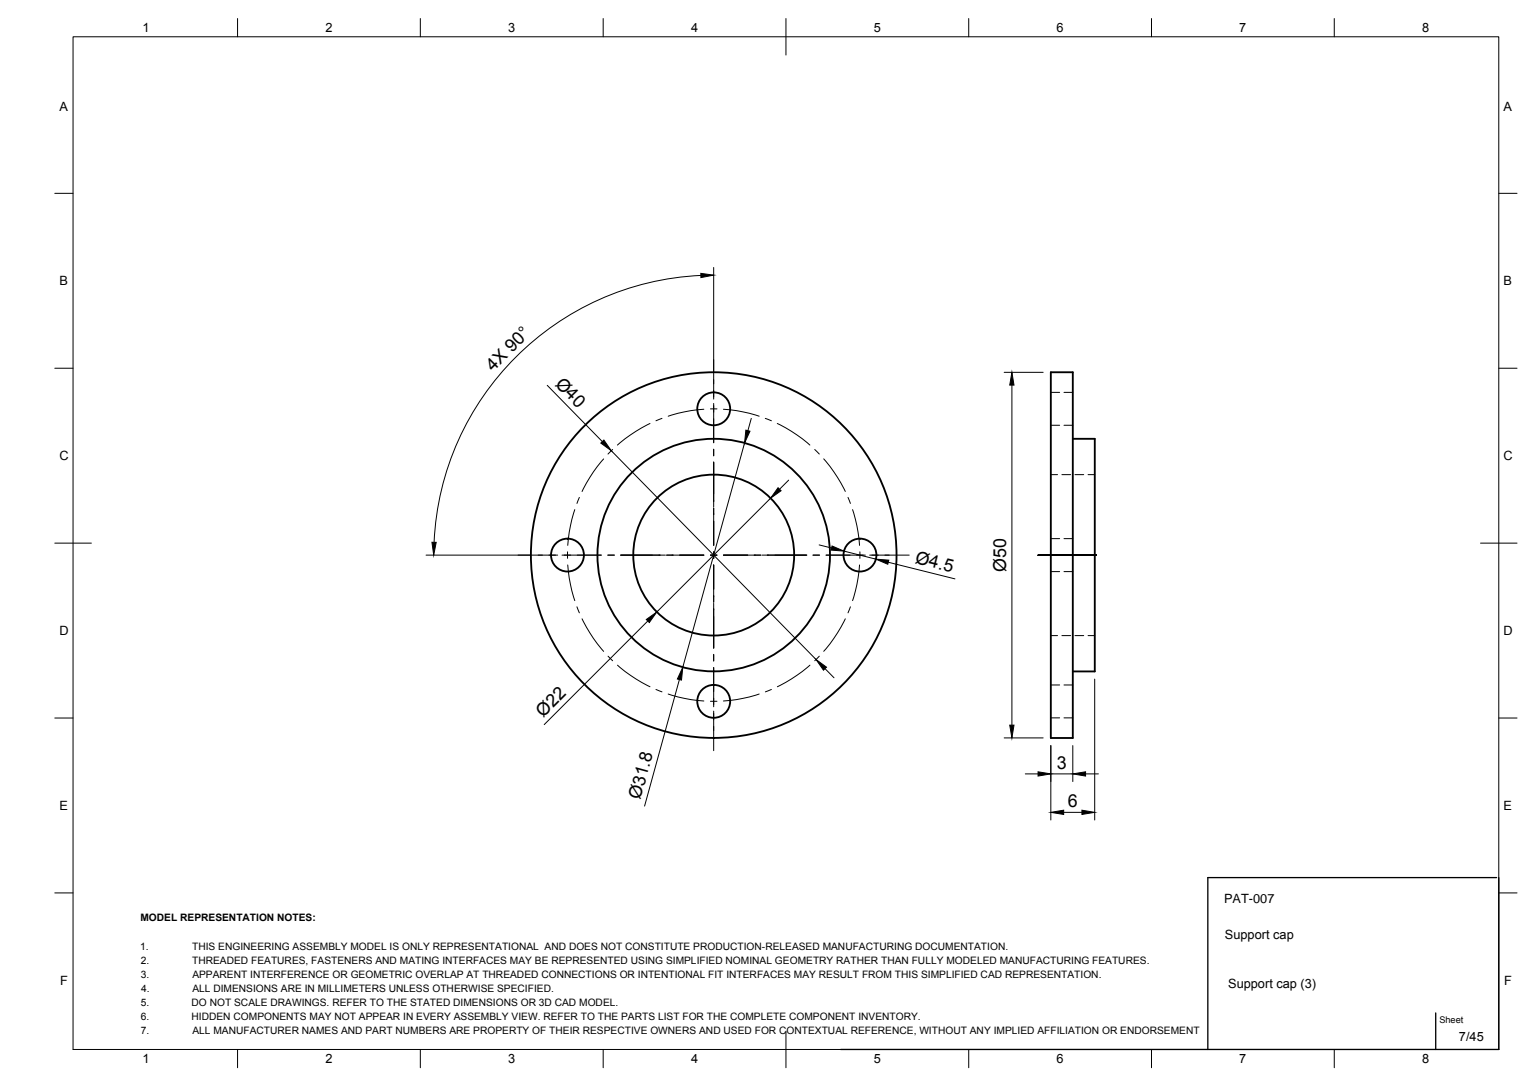
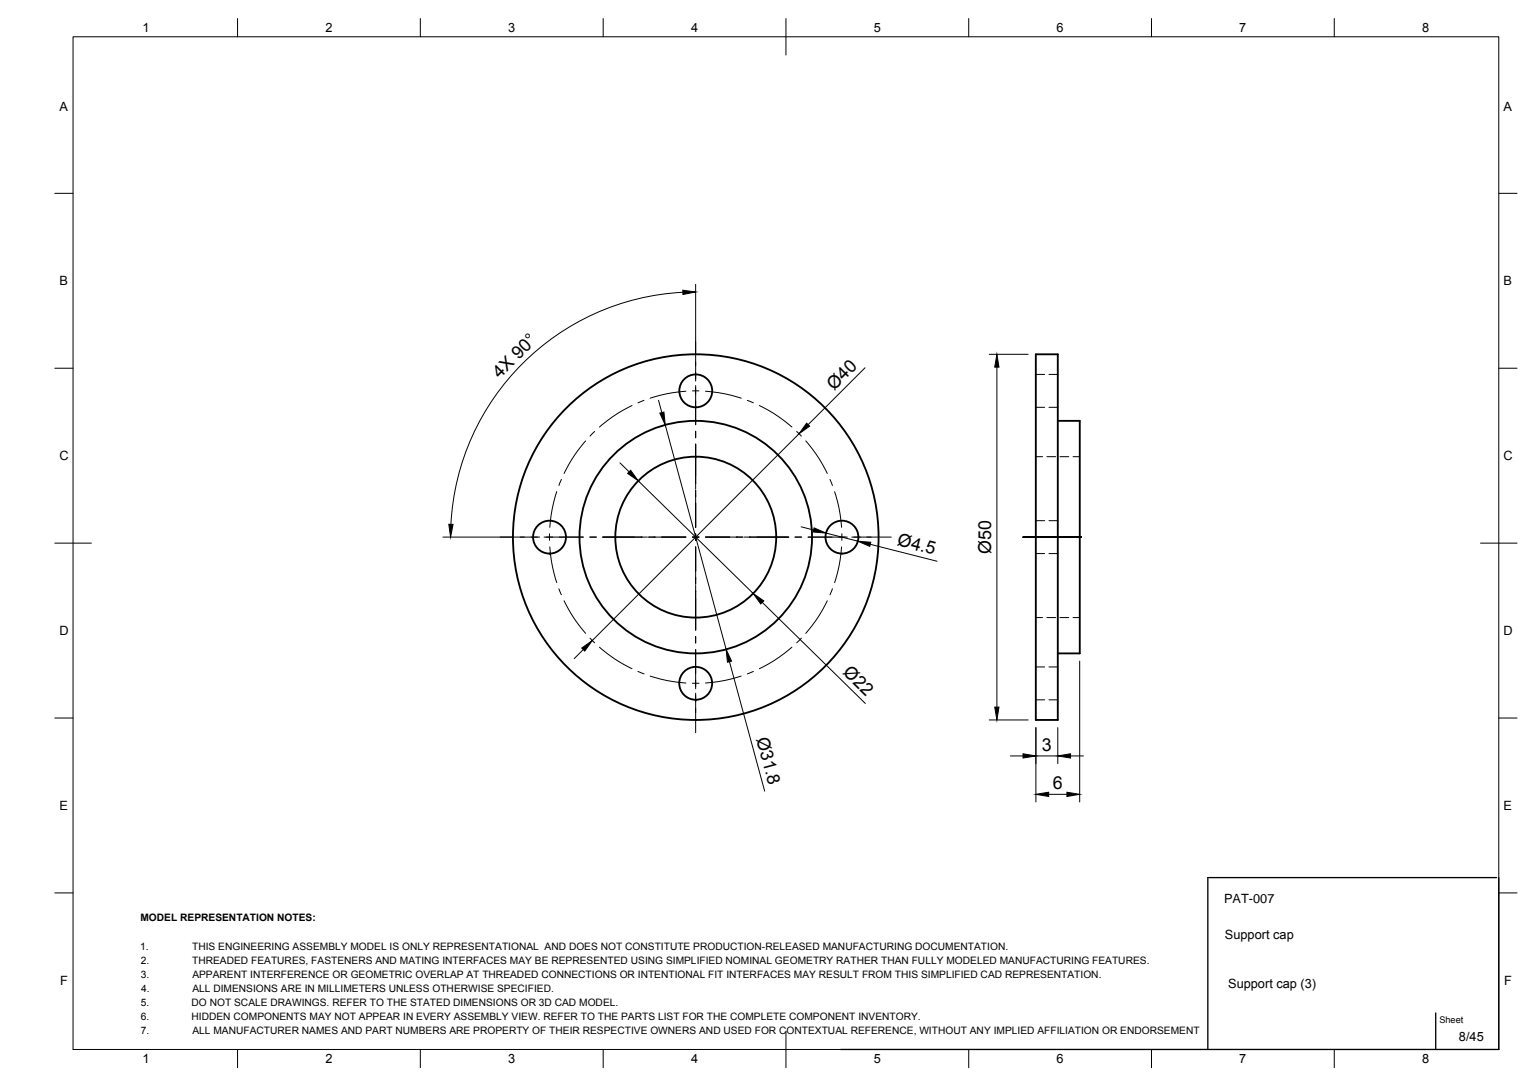
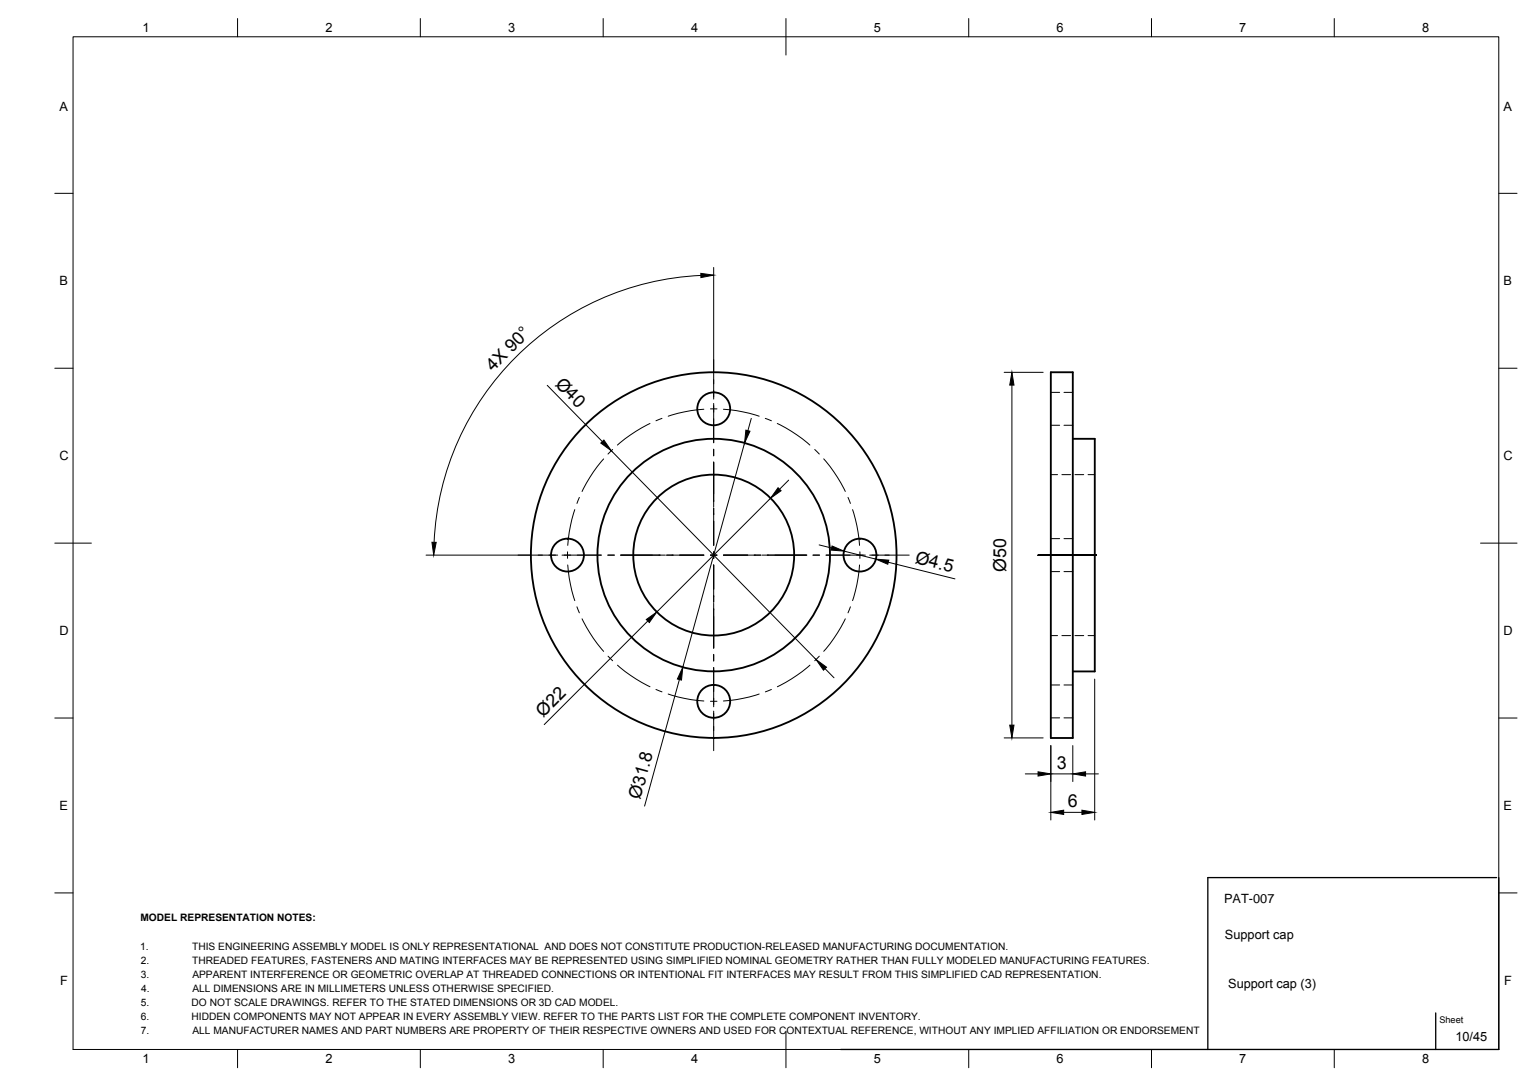
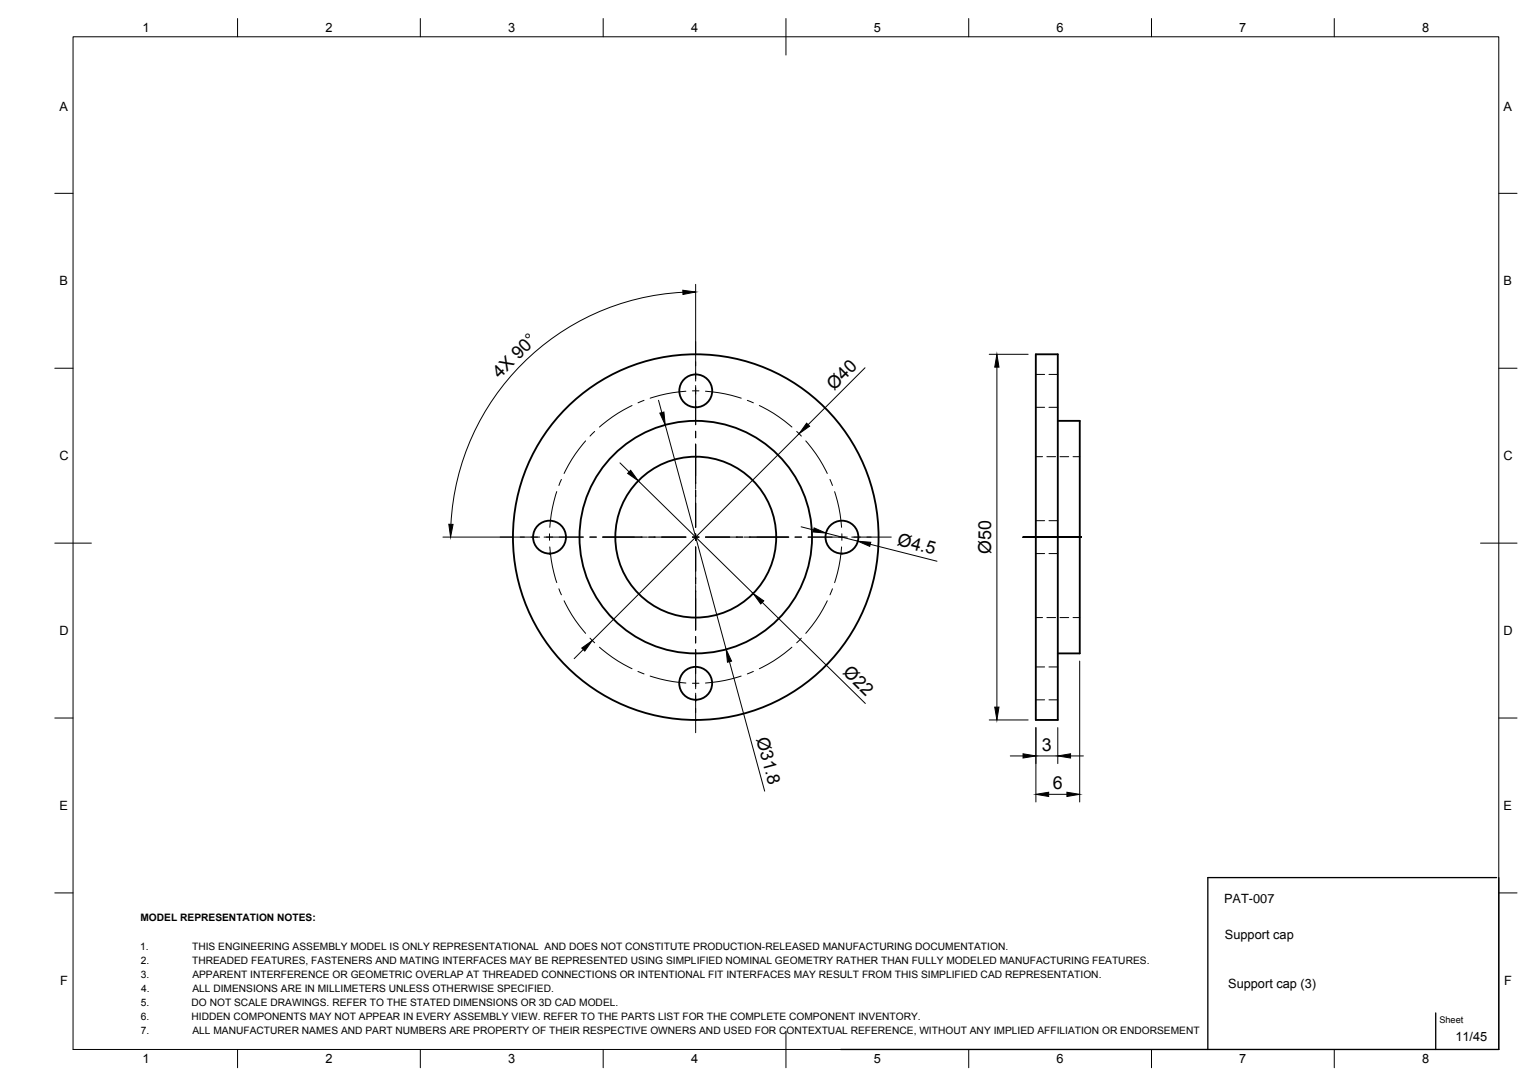
ISO-10303-21;
HEADER;
/* Generated by software containing ST-Developer
 * from STEP Tools, Inc. (www.steptools.com) 
 */

FILE_DESCRIPTION(
/* description */ ('Bearing friction torque test rig'),
/* implementation_level */ '2;1');

FILE_NAME(
/* name */ 'Support cap.step',
/* time_stamp */ '2026-10-28T03:24:04-07:00',
/* author */ (''),
/* organization */ (''),
/* preprocessor_version */ 'ST-DEVELOPER v20.2',
/* originating_system */ 'Autodesk Translation Framework v15.17.0.0',
/* authorisation */ '');

FILE_SCHEMA (('AUTOMOTIVE_DESIGN { 1 0 10303 214 3 1 1 }'));
ENDSEC;

DATA;
#10=MECHANICAL_DESIGN_GEOMETRIC_PRESENTATION_REPRESENTATION('',(#541),#14822);
#463=SHAPE_REPRESENTATION_RELATIONSHIP('SRR','None',#15002,#502);
#502=ADVANCED_BREP_SHAPE_REPRESENTATION('',(#595),#14782);
#541=STYLED_ITEM('',(#15277),#595);
#595=MANIFOLD_SOLID_BREP('Body1',#7657);
#684=FACE_BOUND('',#1629,.T.);
#685=FACE_BOUND('',#1633,.T.);
#686=FACE_BOUND('',#1634,.T.);
#687=FACE_BOUND('',#1635,.T.);
#688=FACE_BOUND('',#1636,.T.);
#689=FACE_BOUND('',#1637,.T.);
#690=FACE_BOUND('',#1639,.T.);
#691=FACE_BOUND('',#1640,.T.);
#692=FACE_BOUND('',#1641,.T.);
#693=FACE_BOUND('',#1642,.T.);
#694=FACE_BOUND('',#1643,.T.);
#891=PLANE('',#8249);
#892=PLANE('',#8256);
#893=PLANE('',#8257);
#1138=FACE_OUTER_BOUND('',#1623,.T.);
#1139=FACE_OUTER_BOUND('',#1624,.T.);
#1140=FACE_OUTER_BOUND('',#1625,.T.);
#1141=FACE_OUTER_BOUND('',#1626,.T.);
#1142=FACE_OUTER_BOUND('',#1627,.T.);
#1143=FACE_OUTER_BOUND('',#1628,.T.);
#1144=FACE_OUTER_BOUND('',#1630,.T.);
#1145=FACE_OUTER_BOUND('',#1631,.T.);
#1146=FACE_OUTER_BOUND('',#1632,.T.);
#1147=FACE_OUTER_BOUND('',#1638,.T.);
#1623=EDGE_LOOP('',(#5346,#5347,#5348,#5349));
#1624=EDGE_LOOP('',(#5350,#5351,#5352,#5353));
#1625=EDGE_LOOP('',(#5354,#5355,#5356,#5357));
#1626=EDGE_LOOP('',(#5358,#5359,#5360,#5361));
#1627=EDGE_LOOP('',(#5362,#5363,#5364,#5365));
#1628=EDGE_LOOP('',(#5366));
#1629=EDGE_LOOP('',(#5367));
#1630=EDGE_LOOP('',(#5368,#5369,#5370,#5371));
#1631=EDGE_LOOP('',(#5372,#5373,#5374,#5375));
#1632=EDGE_LOOP('',(#5376));
#1633=EDGE_LOOP('',(#5377));
#1634=EDGE_LOOP('',(#5378));
#1635=EDGE_LOOP('',(#5379));
#1636=EDGE_LOOP('',(#5380));
#1637=EDGE_LOOP('',(#5381));
#1638=EDGE_LOOP('',(#5382));
#1639=EDGE_LOOP('',(#5383));
#1640=EDGE_LOOP('',(#5384));
#1641=EDGE_LOOP('',(#5385));
#1642=EDGE_LOOP('',(#5386));
#1643=EDGE_LOOP('',(#5387));
#2270=LINE('',#11871,#2714);
#2271=LINE('',#11877,#2715);
#2272=LINE('',#11883,#2716);
#2273=LINE('',#11889,#2717);
#2274=LINE('',#11895,#2718);
#2275=LINE('',#11902,#2719);
#2276=LINE('',#11908,#2720);
#2714=VECTOR('',#9405,0.225);
#2715=VECTOR('',#9412,0.225);
#2716=VECTOR('',#9419,0.225);
#2717=VECTOR('',#9426,0.225);
#2718=VECTOR('',#9433,1.59);
#2719=VECTOR('',#9442,1.1);
#2720=VECTOR('',#9449,2.5);
#3152=CIRCLE('',#8235,0.225);
#3153=CIRCLE('',#8236,0.225);
#3154=CIRCLE('',#8238,0.225);
#3155=CIRCLE('',#8239,0.225);
#3156=CIRCLE('',#8241,0.225);
#3157=CIRCLE('',#8242,0.225);
#3158=CIRCLE('',#8244,0.225);
#3159=CIRCLE('',#8245,0.225);
#3160=CIRCLE('',#8247,1.59);
#3161=CIRCLE('',#8248,1.59);
#3162=CIRCLE('',#8250,1.1);
#3163=CIRCLE('',#8252,1.1);
#3164=CIRCLE('',#8254,2.5);
#3165=CIRCLE('',#8255,2.5);
#3619=VERTEX_POINT('',#11868);
#3620=VERTEX_POINT('',#11870);
#3621=VERTEX_POINT('',#11874);
#3622=VERTEX_POINT('',#11876);
#3623=VERTEX_POINT('',#11880);
#3624=VERTEX_POINT('',#11882);
#3625=VERTEX_POINT('',#11886);
#3626=VERTEX_POINT('',#11888);
#3627=VERTEX_POINT('',#11892);
#3628=VERTEX_POINT('',#11894);
#3629=VERTEX_POINT('',#11898);
#3630=VERTEX_POINT('',#11901);
#3631=VERTEX_POINT('',#11905);
#3632=VERTEX_POINT('',#11907);
#4299=EDGE_CURVE('',#3619,#3619,#3152,.T.);
#4300=EDGE_CURVE('',#3619,#3620,#2270,.T.);
#4301=EDGE_CURVE('',#3620,#3620,#3153,.T.);
#4302=EDGE_CURVE('',#3621,#3621,#3154,.T.);
#4303=EDGE_CURVE('',#3621,#3622,#2271,.T.);
#4304=EDGE_CURVE('',#3622,#3622,#3155,.T.);
#4305=EDGE_CURVE('',#3623,#3623,#3156,.T.);
#4306=EDGE_CURVE('',#3623,#3624,#2272,.T.);
#4307=EDGE_CURVE('',#3624,#3624,#3157,.T.);
#4308=EDGE_CURVE('',#3625,#3625,#3158,.T.);
#4309=EDGE_CURVE('',#3625,#3626,#2273,.T.);
#4310=EDGE_CURVE('',#3626,#3626,#3159,.T.);
#4311=EDGE_CURVE('',#3627,#3627,#3160,.T.);
#4312=EDGE_CURVE('',#3627,#3628,#2274,.T.);
#4313=EDGE_CURVE('',#3628,#3628,#3161,.T.);
#4314=EDGE_CURVE('',#3629,#3629,#3162,.T.);
#4315=EDGE_CURVE('',#3629,#3630,#2275,.T.);
#4316=EDGE_CURVE('',#3630,#3630,#3163,.T.);
#4317=EDGE_CURVE('',#3631,#3631,#3164,.T.);
#4318=EDGE_CURVE('',#3631,#3632,#2276,.T.);
#4319=EDGE_CURVE('',#3632,#3632,#3165,.T.);
#5346=ORIENTED_EDGE('',*,*,#4299,.F.);
#5347=ORIENTED_EDGE('',*,*,#4300,.T.);
#5348=ORIENTED_EDGE('',*,*,#4301,.F.);
#5349=ORIENTED_EDGE('',*,*,#4300,.F.);
#5350=ORIENTED_EDGE('',*,*,#4302,.F.);
#5351=ORIENTED_EDGE('',*,*,#4303,.T.);
#5352=ORIENTED_EDGE('',*,*,#4304,.F.);
#5353=ORIENTED_EDGE('',*,*,#4303,.F.);
#5354=ORIENTED_EDGE('',*,*,#4305,.F.);
#5355=ORIENTED_EDGE('',*,*,#4306,.T.);
#5356=ORIENTED_EDGE('',*,*,#4307,.F.);
#5357=ORIENTED_EDGE('',*,*,#4306,.F.);
#5358=ORIENTED_EDGE('',*,*,#4308,.F.);
#5359=ORIENTED_EDGE('',*,*,#4309,.T.);
#5360=ORIENTED_EDGE('',*,*,#4310,.F.);
#5361=ORIENTED_EDGE('',*,*,#4309,.F.);
#5362=ORIENTED_EDGE('',*,*,#4311,.F.);
#5363=ORIENTED_EDGE('',*,*,#4312,.T.);
#5364=ORIENTED_EDGE('',*,*,#4313,.F.);
#5365=ORIENTED_EDGE('',*,*,#4312,.F.);
#5366=ORIENTED_EDGE('',*,*,#4311,.T.);
#5367=ORIENTED_EDGE('',*,*,#4314,.T.);
#5368=ORIENTED_EDGE('',*,*,#4314,.F.);
#5369=ORIENTED_EDGE('',*,*,#4315,.T.);
#5370=ORIENTED_EDGE('',*,*,#4316,.T.);
#5371=ORIENTED_EDGE('',*,*,#4315,.F.);
#5372=ORIENTED_EDGE('',*,*,#4317,.F.);
#5373=ORIENTED_EDGE('',*,*,#4318,.T.);
#5374=ORIENTED_EDGE('',*,*,#4319,.T.);
#5375=ORIENTED_EDGE('',*,*,#4318,.F.);
#5376=ORIENTED_EDGE('',*,*,#4317,.T.);
#5377=ORIENTED_EDGE('',*,*,#4313,.T.);
#5378=ORIENTED_EDGE('',*,*,#4310,.T.);
#5379=ORIENTED_EDGE('',*,*,#4307,.T.);
#5380=ORIENTED_EDGE('',*,*,#4304,.T.);
#5381=ORIENTED_EDGE('',*,*,#4301,.T.);
#5382=ORIENTED_EDGE('',*,*,#4319,.F.);
#5383=ORIENTED_EDGE('',*,*,#4316,.F.);
#5384=ORIENTED_EDGE('',*,*,#4308,.T.);
#5385=ORIENTED_EDGE('',*,*,#4305,.T.);
#5386=ORIENTED_EDGE('',*,*,#4302,.T.);
#5387=ORIENTED_EDGE('',*,*,#4299,.T.);
#7066=CYLINDRICAL_SURFACE('',#8234,0.225);
#7067=CYLINDRICAL_SURFACE('',#8237,0.225);
#7068=CYLINDRICAL_SURFACE('',#8240,0.225);
#7069=CYLINDRICAL_SURFACE('',#8243,0.225);
#7070=CYLINDRICAL_SURFACE('',#8246,1.59);
#7071=CYLINDRICAL_SURFACE('',#8251,1.1);
#7072=CYLINDRICAL_SURFACE('',#8253,2.5);
#7249=ADVANCED_FACE('',(#1138),#7066,.F.);
#7250=ADVANCED_FACE('',(#1139),#7067,.F.);
#7251=ADVANCED_FACE('',(#1140),#7068,.F.);
#7252=ADVANCED_FACE('',(#1141),#7069,.F.);
#7253=ADVANCED_FACE('',(#1142),#7070,.T.);
#7254=ADVANCED_FACE('',(#1143,#684),#891,.T.);
#7255=ADVANCED_FACE('',(#1144),#7071,.F.);
#7256=ADVANCED_FACE('',(#1145),#7072,.T.);
#7257=ADVANCED_FACE('',(#1146,#685,#686,#687,#688,#689),#892,.T.);
#7258=ADVANCED_FACE('',(#1147,#690,#691,#692,#693,#694),#893,.F.);
#7657=CLOSED_SHELL('',(#7249,#7250,#7251,#7252,#7253,#7254,#7255,#7256,
#7257,#7258));
#8233=AXIS2_PLACEMENT_3D('',#11866,#9399,#9400);
#8234=AXIS2_PLACEMENT_3D('',#11867,#9401,#9402);
#8235=AXIS2_PLACEMENT_3D('',#11869,#9403,#9404);
#8236=AXIS2_PLACEMENT_3D('',#11872,#9406,#9407);
#8237=AXIS2_PLACEMENT_3D('',#11873,#9408,#9409);
#8238=AXIS2_PLACEMENT_3D('',#11875,#9410,#9411);
#8239=AXIS2_PLACEMENT_3D('',#11878,#9413,#9414);
#8240=AXIS2_PLACEMENT_3D('',#11879,#9415,#9416);
#8241=AXIS2_PLACEMENT_3D('',#11881,#9417,#9418);
#8242=AXIS2_PLACEMENT_3D('',#11884,#9420,#9421);
#8243=AXIS2_PLACEMENT_3D('',#11885,#9422,#9423);
#8244=AXIS2_PLACEMENT_3D('',#11887,#9424,#9425);
#8245=AXIS2_PLACEMENT_3D('',#11890,#9427,#9428);
#8246=AXIS2_PLACEMENT_3D('',#11891,#9429,#9430);
#8247=AXIS2_PLACEMENT_3D('',#11893,#9431,#9432);
#8248=AXIS2_PLACEMENT_3D('',#11896,#9434,#9435);
#8249=AXIS2_PLACEMENT_3D('',#11897,#9436,#9437);
#8250=AXIS2_PLACEMENT_3D('',#11899,#9438,#9439);
#8251=AXIS2_PLACEMENT_3D('',#11900,#9440,#9441);
#8252=AXIS2_PLACEMENT_3D('',#11903,#9443,#9444);
#8253=AXIS2_PLACEMENT_3D('',#11904,#9445,#9446);
#8254=AXIS2_PLACEMENT_3D('',#11906,#9447,#9448);
#8255=AXIS2_PLACEMENT_3D('',#11909,#9450,#9451);
#8256=AXIS2_PLACEMENT_3D('',#11910,#9452,#9453);
#8257=AXIS2_PLACEMENT_3D('',#11911,#9454,#9455);
#9399=DIRECTION('axis',(0.,0.,1.));
#9400=DIRECTION('refdir',(1.,0.,0.));
#9401=DIRECTION('center_axis',(0.,1.,0.));
#9402=DIRECTION('ref_axis',(1.,0.,0.));
#9403=DIRECTION('center_axis',(0.,1.,0.));
#9404=DIRECTION('ref_axis',(1.,0.,0.));
#9405=DIRECTION('',(0.,1.,0.));
#9406=DIRECTION('center_axis',(0.,-1.,0.));
#9407=DIRECTION('ref_axis',(1.,0.,0.));
#9408=DIRECTION('center_axis',(0.,1.,0.));
#9409=DIRECTION('ref_axis',(1.,0.,0.));
#9410=DIRECTION('center_axis',(0.,1.,0.));
#9411=DIRECTION('ref_axis',(1.,0.,0.));
#9412=DIRECTION('',(0.,1.,0.));
#9413=DIRECTION('center_axis',(0.,-1.,0.));
#9414=DIRECTION('ref_axis',(1.,0.,0.));
#9415=DIRECTION('center_axis',(0.,1.,0.));
#9416=DIRECTION('ref_axis',(1.,0.,0.));
#9417=DIRECTION('center_axis',(0.,1.,0.));
#9418=DIRECTION('ref_axis',(1.,0.,0.));
#9419=DIRECTION('',(0.,1.,0.));
#9420=DIRECTION('center_axis',(0.,-1.,0.));
#9421=DIRECTION('ref_axis',(1.,0.,0.));
#9422=DIRECTION('center_axis',(0.,1.,0.));
#9423=DIRECTION('ref_axis',(1.,0.,0.));
#9424=DIRECTION('center_axis',(0.,1.,0.));
#9425=DIRECTION('ref_axis',(1.,0.,0.));
#9426=DIRECTION('',(0.,1.,0.));
#9427=DIRECTION('center_axis',(0.,-1.,0.));
#9428=DIRECTION('ref_axis',(1.,0.,0.));
#9429=DIRECTION('center_axis',(0.,1.,0.));
#9430=DIRECTION('ref_axis',(1.,0.,0.));
#9431=DIRECTION('center_axis',(0.,1.,0.));
#9432=DIRECTION('ref_axis',(1.,0.,0.));
#9433=DIRECTION('',(0.,-1.,0.));
#9434=DIRECTION('center_axis',(0.,-1.,0.));
#9435=DIRECTION('ref_axis',(1.,0.,0.));
#9436=DIRECTION('center_axis',(0.,1.,0.));
#9437=DIRECTION('ref_axis',(1.,0.,0.));
#9438=DIRECTION('center_axis',(0.,-1.,0.));
#9439=DIRECTION('ref_axis',(1.,0.,0.));
#9440=DIRECTION('center_axis',(0.,1.,0.));
#9441=DIRECTION('ref_axis',(1.,0.,0.));
#9442=DIRECTION('',(0.,-1.,0.));
#9443=DIRECTION('center_axis',(0.,-1.,0.));
#9444=DIRECTION('ref_axis',(1.,0.,0.));
#9445=DIRECTION('center_axis',(0.,1.,0.));
#9446=DIRECTION('ref_axis',(1.,0.,0.));
#9447=DIRECTION('center_axis',(0.,1.,0.));
#9448=DIRECTION('ref_axis',(1.,0.,0.));
#9449=DIRECTION('',(0.,-1.,0.));
#9450=DIRECTION('center_axis',(0.,1.,0.));
#9451=DIRECTION('ref_axis',(1.,0.,0.));
#9452=DIRECTION('center_axis',(0.,1.,0.));
#9453=DIRECTION('ref_axis',(1.,0.,0.));
#9454=DIRECTION('center_axis',(0.,1.,0.));
#9455=DIRECTION('ref_axis',(1.,0.,0.));
#11866=CARTESIAN_POINT('',(0.,0.,0.));
#11867=CARTESIAN_POINT('Origin',(-2.,-8.2,7.));
#11868=CARTESIAN_POINT('',(-2.225,-8.1,7.));
#11869=CARTESIAN_POINT('Origin',(-2.,-8.1,7.));
#11870=CARTESIAN_POINT('',(-2.225,-7.8,7.));
#11871=CARTESIAN_POINT('',(-2.225,-8.2,7.));
#11872=CARTESIAN_POINT('Origin',(-2.,-7.8,7.));
#11873=CARTESIAN_POINT('Origin',(1.22464679914735E-16,-8.2,9.));
#11874=CARTESIAN_POINT('',(-0.225,-8.1,9.));
#11875=CARTESIAN_POINT('Origin',(1.22464679914735E-16,-8.1,9.));
#11876=CARTESIAN_POINT('',(-0.225,-7.8,9.));
#11877=CARTESIAN_POINT('',(-0.225,-8.2,9.));
#11878=CARTESIAN_POINT('Origin',(1.22464679914735E-16,-7.8,9.));
#11879=CARTESIAN_POINT('Origin',(2.,-8.2,7.));
#11880=CARTESIAN_POINT('',(1.775,-8.1,7.));
#11881=CARTESIAN_POINT('Origin',(2.,-8.1,7.));
#11882=CARTESIAN_POINT('',(1.775,-7.8,7.));
#11883=CARTESIAN_POINT('',(1.775,-8.2,7.));
#11884=CARTESIAN_POINT('Origin',(2.,-7.8,7.));
#11885=CARTESIAN_POINT('Origin',(-3.67394039744206E-16,-8.2,5.));
#11886=CARTESIAN_POINT('',(-0.225,-8.1,5.));
#11887=CARTESIAN_POINT('Origin',(-3.67394039744206E-16,-8.1,5.));
#11888=CARTESIAN_POINT('',(-0.225,-7.8,5.));
#11889=CARTESIAN_POINT('',(-0.225,-8.2,5.));
#11890=CARTESIAN_POINT('Origin',(-3.67394039744206E-16,-7.8,5.));
#11891=CARTESIAN_POINT('Origin',(0.,-7.8,7.));
#11892=CARTESIAN_POINT('',(-1.59,-7.5,7.));
#11893=CARTESIAN_POINT('Origin',(0.,-7.5,7.));
#11894=CARTESIAN_POINT('',(-1.59,-7.8,7.));
#11895=CARTESIAN_POINT('',(-1.59,-7.8,7.));
#11896=CARTESIAN_POINT('Origin',(0.,-7.8,7.));
#11897=CARTESIAN_POINT('Origin',(0.,-7.5,7.));
#11898=CARTESIAN_POINT('',(-1.1,-7.5,7.));
#11899=CARTESIAN_POINT('Origin',(0.,-7.5,7.));
#11900=CARTESIAN_POINT('Origin',(0.,-8.1,7.));
#11901=CARTESIAN_POINT('',(-1.1,-8.1,7.));
#11902=CARTESIAN_POINT('',(-1.1,-8.1,7.));
#11903=CARTESIAN_POINT('Origin',(0.,-8.1,7.));
#11904=CARTESIAN_POINT('Origin',(0.,-8.1,7.));
#11905=CARTESIAN_POINT('',(-2.5,-7.8,7.));
#11906=CARTESIAN_POINT('Origin',(0.,-7.8,7.));
#11907=CARTESIAN_POINT('',(-2.5,-8.1,7.));
#11908=CARTESIAN_POINT('',(-2.5,-8.1,7.));
#11909=CARTESIAN_POINT('Origin',(0.,-8.1,7.));
#11910=CARTESIAN_POINT('Origin',(0.,-7.8,7.));
#11911=CARTESIAN_POINT('Origin',(0.,-8.1,7.));
#14737=UNCERTAINTY_MEASURE_WITH_UNIT(LENGTH_MEASURE(0.001),#14823,
'DISTANCE_ACCURACY_VALUE',
'Maximum model space distance between geometric entities at asserted c
onnectivities');
#14777=UNCERTAINTY_MEASURE_WITH_UNIT(LENGTH_MEASURE(0.001),#14823,
'DISTANCE_ACCURACY_VALUE',
'Maximum model space distance between geometric entities at asserted c
onnectivities');
#14782=(
GEOMETRIC_REPRESENTATION_CONTEXT(3)
GLOBAL_UNCERTAINTY_ASSIGNED_CONTEXT((#14737))
GLOBAL_UNIT_ASSIGNED_CONTEXT((#14823,#14825,#14826))
REPRESENTATION_CONTEXT('','3D')
);
#14822=(
GEOMETRIC_REPRESENTATION_CONTEXT(3)
GLOBAL_UNCERTAINTY_ASSIGNED_CONTEXT((#14777))
GLOBAL_UNIT_ASSIGNED_CONTEXT((#14823,#14825,#14826))
REPRESENTATION_CONTEXT('','3D')
);
#14823=(
LENGTH_UNIT()
NAMED_UNIT(*)
SI_UNIT(.CENTI.,.METRE.)
);
#14825=(
NAMED_UNIT(*)
PLANE_ANGLE_UNIT()
SI_UNIT($,.RADIAN.)
);
#14826=(
NAMED_UNIT(*)
SI_UNIT($,.STERADIAN.)
SOLID_ANGLE_UNIT()
);
#14831=SHAPE_DEFINITION_REPRESENTATION(#14875,#15002);
#14875=PRODUCT_DEFINITION_SHAPE('',$,#15047);
#15002=SHAPE_REPRESENTATION('',(#8233),#14782);
#15042=PRODUCT_DEFINITION_CONTEXT('part definition',#15176,'design');
#15047=PRODUCT_DEFINITION('Support cap','Support cap',#15091,#15042);
#15091=PRODUCT_DEFINITION_FORMATION('',$,#15182);
#15176=APPLICATION_CONTEXT(
'Core Data for Automotive Mechanical Design Process');
#15177=PRODUCT_CONTEXT('part definition',#15176,'mechanical');
#15182=PRODUCT('Support cap','Support cap','Support cap',(#15177));
#15271=COLOUR_RGB('Sky Blue',0.24,0.69,0.87);
#15272=FILL_AREA_STYLE_COLOUR('',#15271);
#15273=FILL_AREA_STYLE('',(#15272));
#15274=SURFACE_STYLE_FILL_AREA(#15273);
#15275=SURFACE_SIDE_STYLE('',(#15274));
#15276=SURFACE_STYLE_USAGE(.BOTH.,#15275);
#15277=PRESENTATION_STYLE_ASSIGNMENT((#15276));
ENDSEC;
END-ISO-10303-21;
